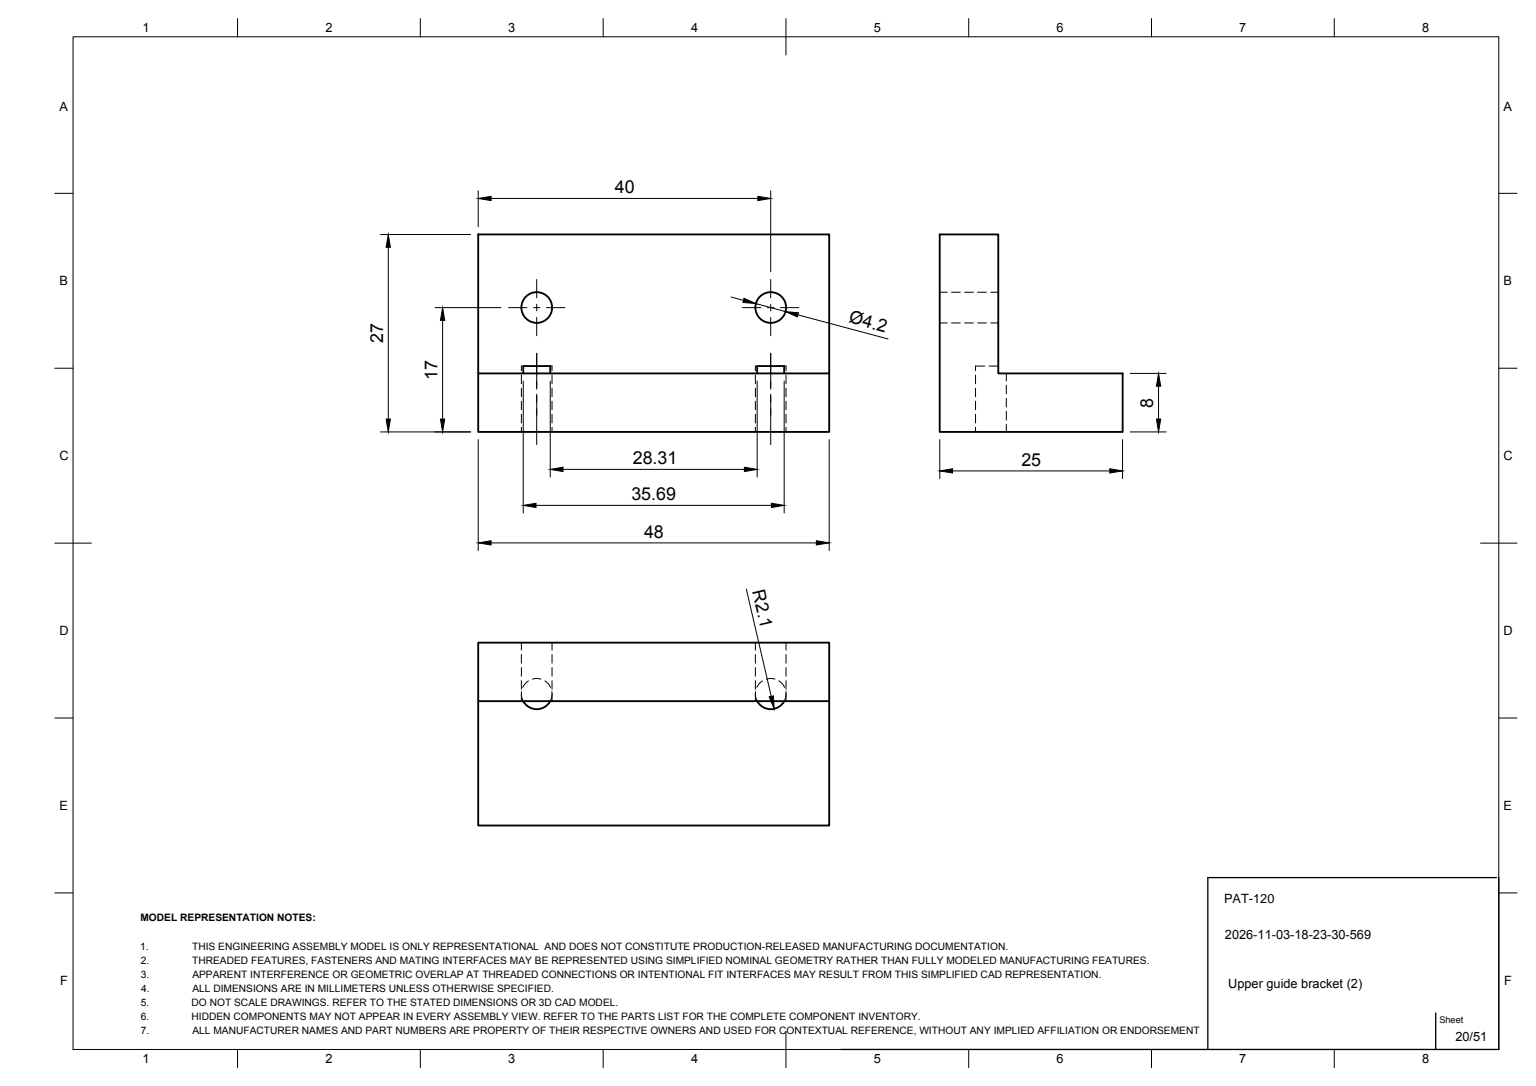
ISO-10303-21;
HEADER;
/* Generated by software containing ST-Developer
 * from STEP Tools, Inc. (www.steptools.com) 
 */

FILE_DESCRIPTION(
/* description */ ('Vibration shaker table dummy'),
/* implementation_level */ '2;1');

FILE_NAME(
/* name */ 'Upper guide bracket (2).step',
/* time_stamp */ '2026-10-27T10:55:14-07:00',
/* author */ (''),
/* organization */ (''),
/* preprocessor_version */ 'ST-DEVELOPER v20.2',
/* originating_system */ 'Autodesk Translation Framework v15.17.0.0',
/* authorisation */ '');

FILE_SCHEMA (('AUTOMOTIVE_DESIGN { 1 0 10303 214 3 1 1 }'));
ENDSEC;

DATA;
#10=MECHANICAL_DESIGN_GEOMETRIC_PRESENTATION_REPRESENTATION('',(#701),#22394);
#609=SHAPE_REPRESENTATION_RELATIONSHIP('SRR','None',#22655,#655);
#655=ADVANCED_BREP_SHAPE_REPRESENTATION('',(#747),#22361);
#701=STYLED_ITEM('',(#22940),#747);
#747=MANIFOLD_SOLID_BREP('Body1',#9219);
#897=FACE_BOUND('',#2139,.T.);
#898=FACE_BOUND('',#2140,.T.);
#899=FACE_BOUND('',#2144,.T.);
#900=FACE_BOUND('',#2145,.T.);
#901=FACE_BOUND('',#2148,.T.);
#902=FACE_BOUND('',#2149,.T.);
#1156=PLANE('',#10113);
#1157=PLANE('',#10119);
#1158=PLANE('',#10120);
#1159=PLANE('',#10121);
#1160=PLANE('',#10122);
#1161=PLANE('',#10123);
#1162=PLANE('',#10124);
#1163=PLANE('',#10125);
#1164=PLANE('',#10126);
#1165=PLANE('',#10127);
#1511=FACE_OUTER_BOUND('',#2131,.T.);
#1512=FACE_OUTER_BOUND('',#2132,.T.);
#1513=FACE_OUTER_BOUND('',#2133,.T.);
#1514=FACE_OUTER_BOUND('',#2134,.T.);
#1515=FACE_OUTER_BOUND('',#2135,.T.);
#1516=FACE_OUTER_BOUND('',#2136,.T.);
#1517=FACE_OUTER_BOUND('',#2137,.T.);
#1518=FACE_OUTER_BOUND('',#2138,.T.);
#1519=FACE_OUTER_BOUND('',#2141,.T.);
#1520=FACE_OUTER_BOUND('',#2142,.T.);
#1521=FACE_OUTER_BOUND('',#2143,.T.);
#1522=FACE_OUTER_BOUND('',#2146,.T.);
#1523=FACE_OUTER_BOUND('',#2147,.T.);
#1524=FACE_OUTER_BOUND('',#2150,.T.);
#2131=EDGE_LOOP('',(#7026,#7027,#7028,#7029));
#2132=EDGE_LOOP('',(#7030,#7031,#7032,#7033));
#2133=EDGE_LOOP('',(#7034,#7035,#7036,#7037,#7038,#7039,#7040,#7041));
#2134=EDGE_LOOP('',(#7042,#7043,#7044));
#2135=EDGE_LOOP('',(#7045,#7046,#7047,#7048,#7049,#7050,#7051,#7052));
#2136=EDGE_LOOP('',(#7053,#7054,#7055));
#2137=EDGE_LOOP('',(#7056,#7057,#7058,#7059,#7060,#7061,#7062,#7063));
#2138=EDGE_LOOP('',(#7064,#7065,#7066,#7067,#7068,#7069,#7070,#7071,#7072,
#7073,#7074,#7075));
#2139=EDGE_LOOP('',(#7076));
#2140=EDGE_LOOP('',(#7077));
#2141=EDGE_LOOP('',(#7078,#7079,#7080,#7081));
#2142=EDGE_LOOP('',(#7082,#7083,#7084,#7085,#7086,#7087));
#2143=EDGE_LOOP('',(#7088,#7089,#7090,#7091));
#2144=EDGE_LOOP('',(#7092));
#2145=EDGE_LOOP('',(#7093));
#2146=EDGE_LOOP('',(#7094,#7095,#7096,#7097,#7098,#7099));
#2147=EDGE_LOOP('',(#7100,#7101,#7102,#7103));
#2148=EDGE_LOOP('',(#7104));
#2149=EDGE_LOOP('',(#7105));
#2150=EDGE_LOOP('',(#7106,#7107,#7108,#7109));
#2854=LINE('',#17658,#3473);
#2855=LINE('',#17664,#3474);
#2856=LINE('',#17670,#3475);
#2857=LINE('',#17674,#3476);
#2858=LINE('',#17678,#3477);
#2859=LINE('',#17681,#3478);
#2860=LINE('',#17686,#3479);
#2861=LINE('',#17690,#3480);
#2862=LINE('',#17694,#3481);
#2863=LINE('',#17697,#3482);
#2864=LINE('',#17699,#3483);
#2865=LINE('',#17701,#3484);
#2866=LINE('',#17703,#3485);
#2867=LINE('',#17705,#3486);
#2868=LINE('',#17707,#3487);
#2869=LINE('',#17708,#3488);
#2870=LINE('',#17711,#3489);
#2871=LINE('',#17713,#3490);
#2872=LINE('',#17714,#3491);
#2873=LINE('',#17718,#3492);
#2874=LINE('',#17719,#3493);
#2875=LINE('',#17720,#3494);
#2876=LINE('',#17724,#3495);
#2877=LINE('',#17725,#3496);
#2878=LINE('',#17726,#3497);
#2879=LINE('',#17730,#3498);
#2880=LINE('',#17731,#3499);
#2881=LINE('',#17732,#3500);
#2882=LINE('',#17734,#3501);
#2883=LINE('',#17735,#3502);
#3473=VECTOR('',#11870,0.21);
#3474=VECTOR('',#11877,0.21);
#3475=VECTOR('',#11884,0.21);
#3476=VECTOR('',#11887,1.);
#3477=VECTOR('',#11890,1.);
#3478=VECTOR('',#11895,1.);
#3479=VECTOR('',#11900,0.21);
#3480=VECTOR('',#11903,1.);
#3481=VECTOR('',#11906,1.);
#3482=VECTOR('',#11911,1.);
#3483=VECTOR('',#11914,1.);
#3484=VECTOR('',#11915,1.);
#3485=VECTOR('',#11916,1.);
#3486=VECTOR('',#11917,1.);
#3487=VECTOR('',#11918,1.);
#3488=VECTOR('',#11919,1.);
#3489=VECTOR('',#11922,1.);
#3490=VECTOR('',#11923,1.);
#3491=VECTOR('',#11924,1.);
#3492=VECTOR('',#11927,1.);
#3493=VECTOR('',#11928,1.);
#3494=VECTOR('',#11929,1.);
#3495=VECTOR('',#11932,1.);
#3496=VECTOR('',#11933,1.);
#3497=VECTOR('',#11934,1.);
#3498=VECTOR('',#11937,1.);
#3499=VECTOR('',#11938,1.);
#3500=VECTOR('',#11939,1.);
#3501=VECTOR('',#11942,1.);
#3502=VECTOR('',#11943,1.);
#4016=CIRCLE('',#10103,0.21);
#4017=CIRCLE('',#10104,0.21);
#4018=CIRCLE('',#10106,0.21);
#4019=CIRCLE('',#10107,0.21);
#4020=CIRCLE('',#10109,0.21);
#4021=CIRCLE('',#10110,0.21);
#4022=CIRCLE('',#10111,0.21);
#4023=CIRCLE('',#10112,0.21);
#4024=CIRCLE('',#10115,0.21);
#4025=CIRCLE('',#10116,0.21);
#4026=CIRCLE('',#10117,0.21);
#4027=CIRCLE('',#10118,0.21);
#4627=VERTEX_POINT('',#17655);
#4628=VERTEX_POINT('',#17657);
#4629=VERTEX_POINT('',#17661);
#4630=VERTEX_POINT('',#17663);
#4631=VERTEX_POINT('',#17667);
#4632=VERTEX_POINT('',#17669);
#4633=VERTEX_POINT('',#17671);
#4634=VERTEX_POINT('',#17673);
#4635=VERTEX_POINT('',#17675);
#4636=VERTEX_POINT('',#17677);
#4637=VERTEX_POINT('',#17683);
#4638=VERTEX_POINT('',#17685);
#4639=VERTEX_POINT('',#17687);
#4640=VERTEX_POINT('',#17689);
#4641=VERTEX_POINT('',#17691);
#4642=VERTEX_POINT('',#17693);
#4643=VERTEX_POINT('',#17700);
#4644=VERTEX_POINT('',#17702);
#4645=VERTEX_POINT('',#17704);
#4646=VERTEX_POINT('',#17706);
#4647=VERTEX_POINT('',#17710);
#4648=VERTEX_POINT('',#17712);
#4649=VERTEX_POINT('',#17716);
#4650=VERTEX_POINT('',#17717);
#4651=VERTEX_POINT('',#17722);
#4652=VERTEX_POINT('',#17723);
#4653=VERTEX_POINT('',#17728);
#4654=VERTEX_POINT('',#17729);
#5506=EDGE_CURVE('',#4627,#4627,#4016,.T.);
#5507=EDGE_CURVE('',#4627,#4628,#2854,.T.);
#5508=EDGE_CURVE('',#4628,#4628,#4017,.T.);
#5509=EDGE_CURVE('',#4629,#4629,#4018,.T.);
#5510=EDGE_CURVE('',#4629,#4630,#2855,.T.);
#5511=EDGE_CURVE('',#4630,#4630,#4019,.T.);
#5512=EDGE_CURVE('',#4631,#4631,#4020,.T.);
#5513=EDGE_CURVE('',#4631,#4632,#2856,.T.);
#5514=EDGE_CURVE('',#4632,#4633,#4021,.T.);
#5515=EDGE_CURVE('',#4634,#4633,#2857,.T.);
#5516=EDGE_CURVE('',#4635,#4634,#4022,.T.);
#5517=EDGE_CURVE('',#4636,#4635,#2858,.T.);
#5518=EDGE_CURVE('',#4636,#4632,#4023,.T.);
#5519=EDGE_CURVE('',#4633,#4636,#2859,.T.);
#5520=EDGE_CURVE('',#4637,#4637,#4024,.T.);
#5521=EDGE_CURVE('',#4637,#4638,#2860,.T.);
#5522=EDGE_CURVE('',#4638,#4639,#4025,.T.);
#5523=EDGE_CURVE('',#4640,#4639,#2861,.T.);
#5524=EDGE_CURVE('',#4641,#4640,#4026,.T.);
#5525=EDGE_CURVE('',#4642,#4641,#2862,.T.);
#5526=EDGE_CURVE('',#4642,#4638,#4027,.T.);
#5527=EDGE_CURVE('',#4639,#4642,#2863,.T.);
#5528=EDGE_CURVE('',#4634,#4641,#2864,.T.);
#5529=EDGE_CURVE('',#4640,#4643,#2865,.T.);
#5530=EDGE_CURVE('',#4644,#4643,#2866,.T.);
#5531=EDGE_CURVE('',#4644,#4645,#2867,.T.);
#5532=EDGE_CURVE('',#4645,#4646,#2868,.T.);
#5533=EDGE_CURVE('',#4646,#4635,#2869,.T.);
#5534=EDGE_CURVE('',#4646,#4647,#2870,.T.);
#5535=EDGE_CURVE('',#4648,#4647,#2871,.T.);
#5536=EDGE_CURVE('',#4643,#4648,#2872,.T.);
#5537=EDGE_CURVE('',#4649,#4650,#2873,.T.);
#5538=EDGE_CURVE('',#4650,#4648,#2874,.T.);
#5539=EDGE_CURVE('',#4647,#4649,#2875,.T.);
#5540=EDGE_CURVE('',#4651,#4652,#2876,.T.);
#5541=EDGE_CURVE('',#4651,#4644,#2877,.T.);
#5542=EDGE_CURVE('',#4652,#4650,#2878,.T.);
#5543=EDGE_CURVE('',#4653,#4654,#2879,.T.);
#5544=EDGE_CURVE('',#4653,#4651,#2880,.T.);
#5545=EDGE_CURVE('',#4654,#4652,#2881,.T.);
#5546=EDGE_CURVE('',#4645,#4653,#2882,.T.);
#5547=EDGE_CURVE('',#4654,#4649,#2883,.T.);
#7026=ORIENTED_EDGE('',*,*,#5506,.F.);
#7027=ORIENTED_EDGE('',*,*,#5507,.T.);
#7028=ORIENTED_EDGE('',*,*,#5508,.F.);
#7029=ORIENTED_EDGE('',*,*,#5507,.F.);
#7030=ORIENTED_EDGE('',*,*,#5509,.F.);
#7031=ORIENTED_EDGE('',*,*,#5510,.T.);
#7032=ORIENTED_EDGE('',*,*,#5511,.F.);
#7033=ORIENTED_EDGE('',*,*,#5510,.F.);
#7034=ORIENTED_EDGE('',*,*,#5512,.F.);
#7035=ORIENTED_EDGE('',*,*,#5513,.T.);
#7036=ORIENTED_EDGE('',*,*,#5514,.T.);
#7037=ORIENTED_EDGE('',*,*,#5515,.F.);
#7038=ORIENTED_EDGE('',*,*,#5516,.F.);
#7039=ORIENTED_EDGE('',*,*,#5517,.F.);
#7040=ORIENTED_EDGE('',*,*,#5518,.T.);
#7041=ORIENTED_EDGE('',*,*,#5513,.F.);
#7042=ORIENTED_EDGE('',*,*,#5519,.F.);
#7043=ORIENTED_EDGE('',*,*,#5514,.F.);
#7044=ORIENTED_EDGE('',*,*,#5518,.F.);
#7045=ORIENTED_EDGE('',*,*,#5520,.F.);
#7046=ORIENTED_EDGE('',*,*,#5521,.T.);
#7047=ORIENTED_EDGE('',*,*,#5522,.T.);
#7048=ORIENTED_EDGE('',*,*,#5523,.F.);
#7049=ORIENTED_EDGE('',*,*,#5524,.F.);
#7050=ORIENTED_EDGE('',*,*,#5525,.F.);
#7051=ORIENTED_EDGE('',*,*,#5526,.T.);
#7052=ORIENTED_EDGE('',*,*,#5521,.F.);
#7053=ORIENTED_EDGE('',*,*,#5527,.F.);
#7054=ORIENTED_EDGE('',*,*,#5522,.F.);
#7055=ORIENTED_EDGE('',*,*,#5526,.F.);
#7056=ORIENTED_EDGE('',*,*,#5516,.T.);
#7057=ORIENTED_EDGE('',*,*,#5528,.T.);
#7058=ORIENTED_EDGE('',*,*,#5524,.T.);
#7059=ORIENTED_EDGE('',*,*,#5529,.T.);
#7060=ORIENTED_EDGE('',*,*,#5530,.F.);
#7061=ORIENTED_EDGE('',*,*,#5531,.T.);
#7062=ORIENTED_EDGE('',*,*,#5532,.T.);
#7063=ORIENTED_EDGE('',*,*,#5533,.T.);
#7064=ORIENTED_EDGE('',*,*,#5517,.T.);
#7065=ORIENTED_EDGE('',*,*,#5533,.F.);
#7066=ORIENTED_EDGE('',*,*,#5534,.T.);
#7067=ORIENTED_EDGE('',*,*,#5535,.F.);
#7068=ORIENTED_EDGE('',*,*,#5536,.F.);
#7069=ORIENTED_EDGE('',*,*,#5529,.F.);
#7070=ORIENTED_EDGE('',*,*,#5523,.T.);
#7071=ORIENTED_EDGE('',*,*,#5527,.T.);
#7072=ORIENTED_EDGE('',*,*,#5525,.T.);
#7073=ORIENTED_EDGE('',*,*,#5528,.F.);
#7074=ORIENTED_EDGE('',*,*,#5515,.T.);
#7075=ORIENTED_EDGE('',*,*,#5519,.T.);
#7076=ORIENTED_EDGE('',*,*,#5506,.T.);
#7077=ORIENTED_EDGE('',*,*,#5509,.T.);
#7078=ORIENTED_EDGE('',*,*,#5537,.T.);
#7079=ORIENTED_EDGE('',*,*,#5538,.T.);
#7080=ORIENTED_EDGE('',*,*,#5535,.T.);
#7081=ORIENTED_EDGE('',*,*,#5539,.T.);
#7082=ORIENTED_EDGE('',*,*,#5540,.F.);
#7083=ORIENTED_EDGE('',*,*,#5541,.T.);
#7084=ORIENTED_EDGE('',*,*,#5530,.T.);
#7085=ORIENTED_EDGE('',*,*,#5536,.T.);
#7086=ORIENTED_EDGE('',*,*,#5538,.F.);
#7087=ORIENTED_EDGE('',*,*,#5542,.F.);
#7088=ORIENTED_EDGE('',*,*,#5543,.F.);
#7089=ORIENTED_EDGE('',*,*,#5544,.T.);
#7090=ORIENTED_EDGE('',*,*,#5540,.T.);
#7091=ORIENTED_EDGE('',*,*,#5545,.F.);
#7092=ORIENTED_EDGE('',*,*,#5512,.T.);
#7093=ORIENTED_EDGE('',*,*,#5520,.T.);
#7094=ORIENTED_EDGE('',*,*,#5532,.F.);
#7095=ORIENTED_EDGE('',*,*,#5546,.T.);
#7096=ORIENTED_EDGE('',*,*,#5543,.T.);
#7097=ORIENTED_EDGE('',*,*,#5547,.T.);
#7098=ORIENTED_EDGE('',*,*,#5539,.F.);
#7099=ORIENTED_EDGE('',*,*,#5534,.F.);
#7100=ORIENTED_EDGE('',*,*,#5547,.F.);
#7101=ORIENTED_EDGE('',*,*,#5545,.T.);
#7102=ORIENTED_EDGE('',*,*,#5542,.T.);
#7103=ORIENTED_EDGE('',*,*,#5537,.F.);
#7104=ORIENTED_EDGE('',*,*,#5508,.T.);
#7105=ORIENTED_EDGE('',*,*,#5511,.T.);
#7106=ORIENTED_EDGE('',*,*,#5546,.F.);
#7107=ORIENTED_EDGE('',*,*,#5531,.F.);
#7108=ORIENTED_EDGE('',*,*,#5541,.F.);
#7109=ORIENTED_EDGE('',*,*,#5544,.F.);
#8578=CYLINDRICAL_SURFACE('',#10102,0.21);
#8579=CYLINDRICAL_SURFACE('',#10105,0.21);
#8580=CYLINDRICAL_SURFACE('',#10108,0.21);
#8581=CYLINDRICAL_SURFACE('',#10114,0.21);
#8876=ADVANCED_FACE('',(#1511),#8578,.F.);
#8877=ADVANCED_FACE('',(#1512),#8579,.F.);
#8878=ADVANCED_FACE('',(#1513),#8580,.F.);
#8879=ADVANCED_FACE('',(#1514),#1156,.F.);
#8880=ADVANCED_FACE('',(#1515),#8581,.F.);
#8881=ADVANCED_FACE('',(#1516),#1157,.F.);
#8882=ADVANCED_FACE('',(#1517),#1158,.T.);
#8883=ADVANCED_FACE('',(#1518,#897,#898),#1159,.T.);
#8884=ADVANCED_FACE('',(#1519),#1160,.T.);
#8885=ADVANCED_FACE('',(#1520),#1161,.T.);
#8886=ADVANCED_FACE('',(#1521,#899,#900),#1162,.T.);
#8887=ADVANCED_FACE('',(#1522),#1163,.T.);
#8888=ADVANCED_FACE('',(#1523,#901,#902),#1164,.T.);
#8889=ADVANCED_FACE('',(#1524),#1165,.F.);
#9219=CLOSED_SHELL('',(#8876,#8877,#8878,#8879,#8880,#8881,#8882,#8883,
#8884,#8885,#8886,#8887,#8888,#8889));
#10101=AXIS2_PLACEMENT_3D('',#17653,#11864,#11865);
#10102=AXIS2_PLACEMENT_3D('',#17654,#11866,#11867);
#10103=AXIS2_PLACEMENT_3D('',#17656,#11868,#11869);
#10104=AXIS2_PLACEMENT_3D('',#17659,#11871,#11872);
#10105=AXIS2_PLACEMENT_3D('',#17660,#11873,#11874);
#10106=AXIS2_PLACEMENT_3D('',#17662,#11875,#11876);
#10107=AXIS2_PLACEMENT_3D('',#17665,#11878,#11879);
#10108=AXIS2_PLACEMENT_3D('',#17666,#11880,#11881);
#10109=AXIS2_PLACEMENT_3D('',#17668,#11882,#11883);
#10110=AXIS2_PLACEMENT_3D('',#17672,#11885,#11886);
#10111=AXIS2_PLACEMENT_3D('',#17676,#11888,#11889);
#10112=AXIS2_PLACEMENT_3D('',#17679,#11891,#11892);
#10113=AXIS2_PLACEMENT_3D('',#17680,#11893,#11894);
#10114=AXIS2_PLACEMENT_3D('',#17682,#11896,#11897);
#10115=AXIS2_PLACEMENT_3D('',#17684,#11898,#11899);
#10116=AXIS2_PLACEMENT_3D('',#17688,#11901,#11902);
#10117=AXIS2_PLACEMENT_3D('',#17692,#11904,#11905);
#10118=AXIS2_PLACEMENT_3D('',#17695,#11907,#11908);
#10119=AXIS2_PLACEMENT_3D('',#17696,#11909,#11910);
#10120=AXIS2_PLACEMENT_3D('',#17698,#11912,#11913);
#10121=AXIS2_PLACEMENT_3D('',#17709,#11920,#11921);
#10122=AXIS2_PLACEMENT_3D('',#17715,#11925,#11926);
#10123=AXIS2_PLACEMENT_3D('',#17721,#11930,#11931);
#10124=AXIS2_PLACEMENT_3D('',#17727,#11935,#11936);
#10125=AXIS2_PLACEMENT_3D('',#17733,#11940,#11941);
#10126=AXIS2_PLACEMENT_3D('',#17736,#11944,#11945);
#10127=AXIS2_PLACEMENT_3D('',#17737,#11946,#11947);
#11864=DIRECTION('axis',(0.,0.,1.));
#11865=DIRECTION('refdir',(1.,0.,0.));
#11866=DIRECTION('center_axis',(0.,0.,1.));
#11867=DIRECTION('ref_axis',(1.,0.,0.));
#11868=DIRECTION('center_axis',(0.,0.,1.));
#11869=DIRECTION('ref_axis',(1.,0.,0.));
#11870=DIRECTION('',(0.,0.,1.));
#11871=DIRECTION('center_axis',(0.,0.,-1.));
#11872=DIRECTION('ref_axis',(1.,0.,0.));
#11873=DIRECTION('center_axis',(0.,0.,1.));
#11874=DIRECTION('ref_axis',(1.,0.,0.));
#11875=DIRECTION('center_axis',(0.,0.,1.));
#11876=DIRECTION('ref_axis',(1.,0.,0.));
#11877=DIRECTION('',(0.,0.,1.));
#11878=DIRECTION('center_axis',(0.,0.,-1.));
#11879=DIRECTION('ref_axis',(1.,0.,0.));
#11880=DIRECTION('center_axis',(0.,1.,0.));
#11881=DIRECTION('ref_axis',(1.,0.,0.));
#11882=DIRECTION('center_axis',(0.,1.,0.));
#11883=DIRECTION('ref_axis',(1.,0.,0.));
#11884=DIRECTION('',(0.,1.,0.));
#11885=DIRECTION('center_axis',(0.,1.,0.));
#11886=DIRECTION('ref_axis',(1.,0.,0.));
#11887=DIRECTION('',(0.,1.,0.));
#11888=DIRECTION('center_axis',(0.,-1.,0.));
#11889=DIRECTION('ref_axis',(1.,0.,0.));
#11890=DIRECTION('',(0.,-1.,0.));
#11891=DIRECTION('center_axis',(0.,1.,0.));
#11892=DIRECTION('ref_axis',(1.,0.,0.));
#11893=DIRECTION('center_axis',(0.,1.,0.));
#11894=DIRECTION('ref_axis',(1.,0.,0.));
#11895=DIRECTION('',(-1.,0.,0.));
#11896=DIRECTION('center_axis',(0.,1.,0.));
#11897=DIRECTION('ref_axis',(1.,0.,0.));
#11898=DIRECTION('center_axis',(0.,1.,0.));
#11899=DIRECTION('ref_axis',(1.,0.,0.));
#11900=DIRECTION('',(0.,1.,0.));
#11901=DIRECTION('center_axis',(0.,1.,0.));
#11902=DIRECTION('ref_axis',(1.,0.,0.));
#11903=DIRECTION('',(0.,1.,0.));
#11904=DIRECTION('center_axis',(0.,-1.,0.));
#11905=DIRECTION('ref_axis',(1.,0.,0.));
#11906=DIRECTION('',(0.,-1.,0.));
#11907=DIRECTION('center_axis',(0.,1.,0.));
#11908=DIRECTION('ref_axis',(1.,0.,0.));
#11909=DIRECTION('center_axis',(0.,1.,0.));
#11910=DIRECTION('ref_axis',(1.,0.,0.));
#11911=DIRECTION('',(-1.,0.,0.));
#11912=DIRECTION('center_axis',(0.,1.,0.));
#11913=DIRECTION('ref_axis',(-1.,0.,0.));
#11914=DIRECTION('',(1.,0.,0.));
#11915=DIRECTION('',(1.,0.,0.));
#11916=DIRECTION('',(0.,0.,1.));
#11917=DIRECTION('',(-1.,0.,0.));
#11918=DIRECTION('',(0.,0.,1.));
#11919=DIRECTION('',(1.,0.,0.));
#11920=DIRECTION('center_axis',(0.,0.,-1.));
#11921=DIRECTION('ref_axis',(-1.,0.,0.));
#11922=DIRECTION('',(0.,1.,0.));
#11923=DIRECTION('',(-1.,0.,0.));
#11924=DIRECTION('',(0.,1.,0.));
#11925=DIRECTION('center_axis',(0.,1.,0.));
#11926=DIRECTION('ref_axis',(0.,0.,1.));
#11927=DIRECTION('',(1.,0.,0.));
#11928=DIRECTION('',(0.,0.,-1.));
#11929=DIRECTION('',(0.,0.,1.));
#11930=DIRECTION('center_axis',(1.,0.,0.));
#11931=DIRECTION('ref_axis',(0.,1.,0.));
#11932=DIRECTION('',(0.,0.,1.));
#11933=DIRECTION('',(0.,1.,0.));
#11934=DIRECTION('',(0.,1.,0.));
#11935=DIRECTION('center_axis',(0.,-1.,0.));
#11936=DIRECTION('ref_axis',(1.,0.,0.));
#11937=DIRECTION('',(0.,0.,1.));
#11938=DIRECTION('',(1.,0.,0.));
#11939=DIRECTION('',(1.,0.,0.));
#11940=DIRECTION('center_axis',(-1.,0.,0.));
#11941=DIRECTION('ref_axis',(0.,-1.,0.));
#11942=DIRECTION('',(0.,-1.,0.));
#11943=DIRECTION('',(0.,1.,0.));
#11944=DIRECTION('center_axis',(0.,0.,1.));
#11945=DIRECTION('ref_axis',(1.,0.,0.));
#11946=DIRECTION('center_axis',(0.,0.,1.));
#11947=DIRECTION('ref_axis',(1.,0.,0.));
#17653=CARTESIAN_POINT('',(0.,0.,0.));
#17654=CARTESIAN_POINT('Origin',(4.4,0.,29.6));
#17655=CARTESIAN_POINT('',(4.19,-2.57175827820944E-17,29.7));
#17656=CARTESIAN_POINT('Origin',(4.4,0.,29.7));
#17657=CARTESIAN_POINT('',(4.19,2.57175827820944E-17,30.5));
#17658=CARTESIAN_POINT('',(4.19,-2.57175827820944E-17,29.6));
#17659=CARTESIAN_POINT('Origin',(4.4,0.,30.5));
#17660=CARTESIAN_POINT('Origin',(7.6,0.,29.6));
#17661=CARTESIAN_POINT('',(7.39,-2.57175827820944E-17,29.7));
#17662=CARTESIAN_POINT('Origin',(7.6,0.,29.7));
#17663=CARTESIAN_POINT('',(7.39,2.57175827820944E-17,30.5));
#17664=CARTESIAN_POINT('',(7.39,-2.57175827820944E-17,29.6));
#17665=CARTESIAN_POINT('Origin',(7.6,0.,30.5));
#17666=CARTESIAN_POINT('Origin',(4.4,-1.8,29.8));
#17667=CARTESIAN_POINT('',(4.19,-1.7,29.8));
#17668=CARTESIAN_POINT('Origin',(4.4,-1.7,29.8));
#17669=CARTESIAN_POINT('',(4.19,-0.8,29.8));
#17670=CARTESIAN_POINT('',(4.19,-1.8,29.8));
#17671=CARTESIAN_POINT('',(4.58466185312619,-0.8,29.7));
#17672=CARTESIAN_POINT('Origin',(4.4,-0.8,29.8));
#17673=CARTESIAN_POINT('',(4.5846618531262,-0.9,29.7));
#17674=CARTESIAN_POINT('',(4.58466185312619,-1.8,29.7));
#17675=CARTESIAN_POINT('',(4.21533814687381,-0.9,29.7));
#17676=CARTESIAN_POINT('Origin',(4.4,-0.9,29.8));
#17677=CARTESIAN_POINT('',(4.21533814687381,-0.8,29.7));
#17678=CARTESIAN_POINT('',(4.21533814687381,-1.8,29.7));
#17679=CARTESIAN_POINT('Origin',(4.4,-0.8,29.8));
#17680=CARTESIAN_POINT('Origin',(4.4,-0.8,29.8));
#17681=CARTESIAN_POINT('',(6.4,-0.8,29.7));
#17682=CARTESIAN_POINT('Origin',(7.6,-1.8,29.8));
#17683=CARTESIAN_POINT('',(7.39,-1.7,29.8));
#17684=CARTESIAN_POINT('Origin',(7.6,-1.7,29.8));
#17685=CARTESIAN_POINT('',(7.39,-0.8,29.8));
#17686=CARTESIAN_POINT('',(7.39,-1.8,29.8));
#17687=CARTESIAN_POINT('',(7.78466185312619,-0.8,29.7));
#17688=CARTESIAN_POINT('Origin',(7.6,-0.8,29.8));
#17689=CARTESIAN_POINT('',(7.78466185312619,-0.9,29.7));
#17690=CARTESIAN_POINT('',(7.78466185312619,-1.8,29.7));
#17691=CARTESIAN_POINT('',(7.4153381468738,-0.9,29.7));
#17692=CARTESIAN_POINT('Origin',(7.6,-0.9,29.8));
#17693=CARTESIAN_POINT('',(7.41533814687381,-0.8,29.7));
#17694=CARTESIAN_POINT('',(7.41533814687381,-1.8,29.7));
#17695=CARTESIAN_POINT('Origin',(7.6,-0.8,29.8));
#17696=CARTESIAN_POINT('Origin',(7.6,-0.8,29.8));
#17697=CARTESIAN_POINT('',(8.,-0.8,29.7));
#17698=CARTESIAN_POINT('Origin',(8.4,-0.9,28.));
#17699=CARTESIAN_POINT('',(8.4,-0.9,29.7));
#17700=CARTESIAN_POINT('',(8.4,-0.9,29.7));
#17701=CARTESIAN_POINT('',(8.4,-0.9,29.7));
#17702=CARTESIAN_POINT('',(8.4,-0.9,28.));
#17703=CARTESIAN_POINT('',(8.4,-0.9,28.));
#17704=CARTESIAN_POINT('',(3.6,-0.9,28.));
#17705=CARTESIAN_POINT('',(8.4,-0.9,28.));
#17706=CARTESIAN_POINT('',(3.6,-0.9,29.7));
#17707=CARTESIAN_POINT('',(3.6,-0.9,28.));
#17708=CARTESIAN_POINT('',(8.4,-0.9,29.7));
#17709=CARTESIAN_POINT('Origin',(8.4,-1.7,29.7));
#17710=CARTESIAN_POINT('',(3.6,1.,29.7));
#17711=CARTESIAN_POINT('',(3.6,-1.7,29.7));
#17712=CARTESIAN_POINT('',(8.4,1.,29.7));
#17713=CARTESIAN_POINT('',(3.6,1.,29.7));
#17714=CARTESIAN_POINT('',(8.4,-1.7,29.7));
#17715=CARTESIAN_POINT('Origin',(6.,1.,30.1));
#17716=CARTESIAN_POINT('',(3.6,1.,30.5));
#17717=CARTESIAN_POINT('',(8.4,1.,30.5));
#17718=CARTESIAN_POINT('',(8.4,1.,30.5));
#17719=CARTESIAN_POINT('',(8.4,1.,29.7));
#17720=CARTESIAN_POINT('',(3.6,1.,30.5));
#17721=CARTESIAN_POINT('Origin',(8.4,-1.7,28.));
#17722=CARTESIAN_POINT('',(8.4,-1.7,28.));
#17723=CARTESIAN_POINT('',(8.4,-1.7,30.5));
#17724=CARTESIAN_POINT('',(8.4,-1.7,28.));
#17725=CARTESIAN_POINT('',(8.4,-1.7,28.));
#17726=CARTESIAN_POINT('',(8.4,-1.7,30.5));
#17727=CARTESIAN_POINT('Origin',(3.6,-1.7,28.));
#17728=CARTESIAN_POINT('',(3.6,-1.7,28.));
#17729=CARTESIAN_POINT('',(3.6,-1.7,30.5));
#17730=CARTESIAN_POINT('',(3.6,-1.7,28.));
#17731=CARTESIAN_POINT('',(3.6,-1.7,28.));
#17732=CARTESIAN_POINT('',(3.6,-1.7,30.5));
#17733=CARTESIAN_POINT('Origin',(3.6,-0.9,28.));
#17734=CARTESIAN_POINT('',(3.6,-0.9,28.));
#17735=CARTESIAN_POINT('',(3.6,-1.7,30.5));
#17736=CARTESIAN_POINT('Origin',(6.,-1.3,30.5));
#17737=CARTESIAN_POINT('Origin',(6.,-1.3,28.));
#22310=UNCERTAINTY_MEASURE_WITH_UNIT(LENGTH_MEASURE(0.001),#22395,
'DISTANCE_ACCURACY_VALUE',
'Maximum model space distance between geometric entities at asserted c
onnectivities');
#22343=UNCERTAINTY_MEASURE_WITH_UNIT(LENGTH_MEASURE(0.001),#22395,
'DISTANCE_ACCURACY_VALUE',
'Maximum model space distance between geometric entities at asserted c
onnectivities');
#22361=(
GEOMETRIC_REPRESENTATION_CONTEXT(3)
GLOBAL_UNCERTAINTY_ASSIGNED_CONTEXT((#22310))
GLOBAL_UNIT_ASSIGNED_CONTEXT((#22395,#22397,#22398))
REPRESENTATION_CONTEXT('','3D')
);
#22394=(
GEOMETRIC_REPRESENTATION_CONTEXT(3)
GLOBAL_UNCERTAINTY_ASSIGNED_CONTEXT((#22343))
GLOBAL_UNIT_ASSIGNED_CONTEXT((#22395,#22397,#22398))
REPRESENTATION_CONTEXT('','3D')
);
#22395=(
LENGTH_UNIT()
NAMED_UNIT(*)
SI_UNIT(.CENTI.,.METRE.)
);
#22397=(
NAMED_UNIT(*)
PLANE_ANGLE_UNIT()
SI_UNIT($,.RADIAN.)
);
#22398=(
NAMED_UNIT(*)
SI_UNIT($,.STERADIAN.)
SOLID_ANGLE_UNIT()
);
#22416=SHAPE_DEFINITION_REPRESENTATION(#22466,#22655);
#22466=PRODUCT_DEFINITION_SHAPE('',$,#22706);
#22655=SHAPE_REPRESENTATION('',(#10101),#22361);
#22688=PRODUCT_DEFINITION_CONTEXT('part definition',#22840,'design');
#22706=PRODUCT_DEFINITION('Upper guide bracket (2)',
'Upper guide bracket (2)',#22756,#22688);
#22756=PRODUCT_DEFINITION_FORMATION('',$,#22859);
#22840=APPLICATION_CONTEXT(
'Core Data for Automotive Mechanical Design Process');
#22841=PRODUCT_CONTEXT('part definition',#22840,'mechanical');
#22859=PRODUCT('Upper guide bracket (2)','Upper guide bracket (2)',
'Upper guide bracket (2)',(#22841));
#22934=COLOUR_RGB('Dark Blue',0.08,0.2,0.34);
#22935=FILL_AREA_STYLE_COLOUR('',#22934);
#22936=FILL_AREA_STYLE('',(#22935));
#22937=SURFACE_STYLE_FILL_AREA(#22936);
#22938=SURFACE_SIDE_STYLE('',(#22937));
#22939=SURFACE_STYLE_USAGE(.BOTH.,#22938);
#22940=PRESENTATION_STYLE_ASSIGNMENT((#22939));
ENDSEC;
END-ISO-10303-21;
